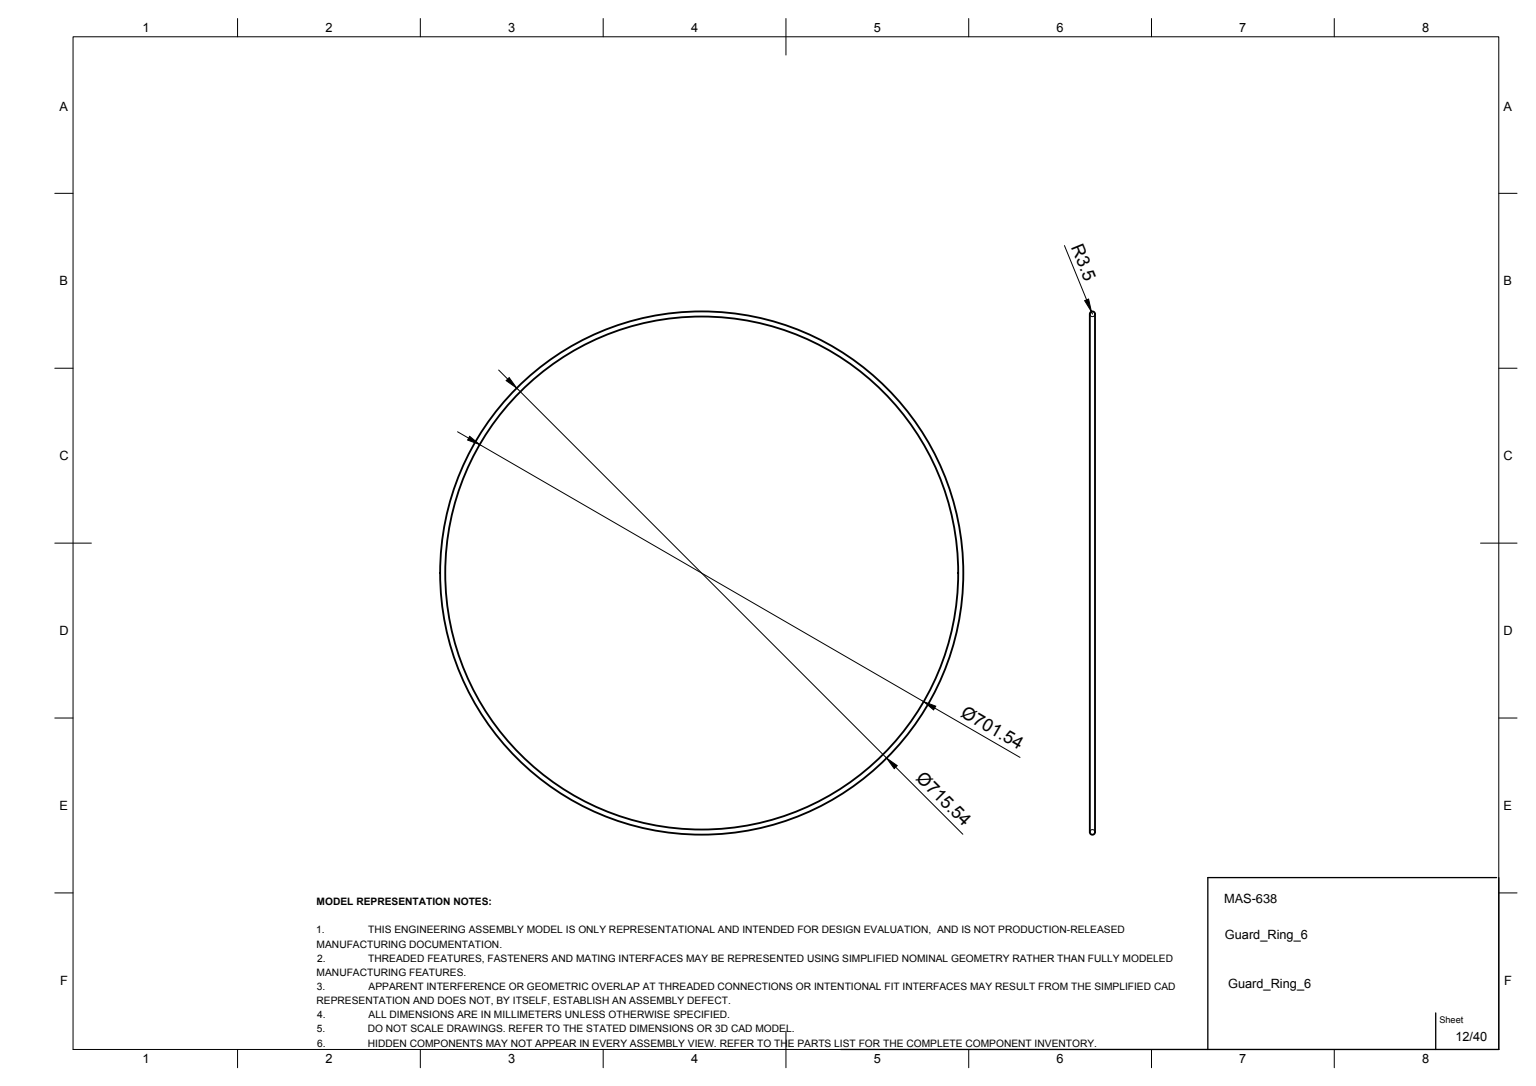
ISO-10303-21;
HEADER;
FILE_DESCRIPTION((''),'2;1');
FILE_NAME('Guard_Ring_6.step','2026-10-09T12:00:21-07:00',(''),(''),'','','');
FILE_SCHEMA (('AUTOMOTIVE_DESIGN { 1 0 10303 214 3 1 1 }'));
ENDSEC;
DATA;
#10=MECHANICAL_DESIGN_GEOMETRIC_PRESENTATION_REPRESENTATION('',(#403),#10334);
#339=SHAPE_REPRESENTATION_RELATIONSHIP('SRR','None',#10455,#371) ;
#371=ADVANCED_BREP_SHAPE_REPRESENTATION('',(#443),#10307) ;
#403=STYLED_ITEM('',(#10631),#443) ;
#443=MANIFOLD_SOLID_BREP('Body1',#3565) ;
#864=FACE_OUTER_BOUND('',#1064,.T.) ;
#1064=EDGE_LOOP('',(#2369,#2370,#2371,#2372)) ;
#1286=CIRCLE('',#3995,0.349999999999999) ;
#1287=CIRCLE('',#3996,35.0768144613668) ;
#1518=VERTEX_POINT('',#5678) ;
#1841=EDGE_CURVE('',#1518,#1518,#1286,.T.) ;
#1842=EDGE_CURVE('',#1518,#1518,#1287,.T.) ;
#2369=ORIENTED_EDGE('',*,*,#1841,.F.) ;
#2370=ORIENTED_EDGE('',*,*,#1842,.T.) ;
#2371=ORIENTED_EDGE('',*,*,#1841,.T.) ;
#2372=ORIENTED_EDGE('',*,*,#1842,.F.) ;
#3310=TOROIDAL_SURFACE('',#3994,35.4268144613668,0.349999999999999) ;
#3372=ADVANCED_FACE('',(#864),#3310,.T.) ;
#3565=CLOSED_SHELL('',(#3372)) ;
#3993=AXIS2_PLACEMENT_3D('',#5676,#4547,#4548) ;
#3994=AXIS2_PLACEMENT_3D('',#5677,#4549,#4550) ;
#3995=AXIS2_PLACEMENT_3D('',#5679,#4551,#4552) ;
#3996=AXIS2_PLACEMENT_3D('',#5680,#4553,#4554) ;
#4547=DIRECTION('axis',(0.,0.,1.)) ;
#4548=DIRECTION('refdir',(1.,0.,0.)) ;
#4549=DIRECTION('center_axis',(-6.42891162084177E-17,-1.,-1.01883556321148E-16)) ;
#4550=DIRECTION('ref_axis',(1.,0.,0.)) ;
#4551=DIRECTION('center_axis',(0.,1.01883556321148E-16,-1.)) ;
#4552=DIRECTION('ref_axis',(-1.,0.,0.)) ;
#4553=DIRECTION('center_axis',(6.42891162084177E-17,1.,1.01883556321148E-16)) ;
#4554=DIRECTION('ref_axis',(1.,-6.42891162084177E-17,-6.55000379205715E-33)) ;
#5676=CARTESIAN_POINT('',(0.,0.,0.)) ;
#5677=CARTESIAN_POINT('Origin',(23.47768801576,67.3831179463143,68.2224337400009)) ;
#5678=CARTESIAN_POINT('',(-11.5991264456068,67.3831179463143,68.2224337400009)) ;
#5679=CARTESIAN_POINT('Origin',(-11.9491264456068,67.3831179463143,68.2224337400009)) ;
#5680=CARTESIAN_POINT('Origin',(23.47768801576,67.3831179463143,68.2224337400009)) ;
#10270=UNCERTAINTY_MEASURE_WITH_UNIT(LENGTH_MEASURE(0.001),#10335,
'DISTANCE_ACCURACY_VALUE',
'Maximum model space distance between geometric entities at asserted c
onnectivities') ;
#10297=UNCERTAINTY_MEASURE_WITH_UNIT(LENGTH_MEASURE(0.001),#10335,
'DISTANCE_ACCURACY_VALUE',
'Maximum model space distance between geometric entities at asserted c
onnectivities') ;
#10307=(
GEOMETRIC_REPRESENTATION_CONTEXT(3)
GLOBAL_UNCERTAINTY_ASSIGNED_CONTEXT((#10270))
GLOBAL_UNIT_ASSIGNED_CONTEXT((#10335,#10337,#10338))
REPRESENTATION_CONTEXT('','3D')
) ;
#10334=(
GEOMETRIC_REPRESENTATION_CONTEXT(3)
GLOBAL_UNCERTAINTY_ASSIGNED_CONTEXT((#10297))
GLOBAL_UNIT_ASSIGNED_CONTEXT((#10335,#10337,#10338))
REPRESENTATION_CONTEXT('','3D')
) ;
#10335=(
LENGTH_UNIT()
NAMED_UNIT(*)
SI_UNIT(.CENTI.,.METRE.)
) ;
#10337=(
NAMED_UNIT(*)
PLANE_ANGLE_UNIT()
SI_UNIT($,.RADIAN.)
) ;
#10338=(
NAMED_UNIT(*)
SI_UNIT($,.STERADIAN.)
SOLID_ANGLE_UNIT()
) ;
#10348=SHAPE_DEFINITION_REPRESENTATION(#10384,#10455) ;
#10384=PRODUCT_DEFINITION_SHAPE('',$,#10492) ;
#10455=SHAPE_REPRESENTATION('',(#3993),#10307) ;
#10482=PRODUCT_DEFINITION_CONTEXT('part definition',#10592,'design') ;
#10492=PRODUCT_DEFINITION('Guard_Ring_6','Guard_Ring_6',#10528,#10482) ;
#10528=PRODUCT_DEFINITION_FORMATION('',$,#10603) ;
#10592=APPLICATION_CONTEXT(
'Core Data for Automotive Mechanical Design Process') ;
#10593=PRODUCT_CONTEXT('part definition',#10592,'mechanical') ;
#10603=PRODUCT('Guard_Ring_6','Guard_Ring_6',$,(#10593)) ;
#10631=PRESENTATION_STYLE_ASSIGNMENT((#10635)) ;
#10635=SURFACE_STYLE_USAGE(.BOTH.,#10639) ;
#10639=SURFACE_SIDE_STYLE('',(#10643)) ;
#10643=SURFACE_STYLE_FILL_AREA(#10647) ;
#10647=FILL_AREA_STYLE('Opaque(25,25,25)',(#10651)) ;
#10651=FILL_AREA_STYLE_COLOUR('Opaque(25,25,25)',#10655) ;
#10655=COLOUR_RGB('Opaque(25,25,25)', 0.09019608, 0.27058824, 0.51372549) ;
ENDSEC;
END-ISO-10303-21;
